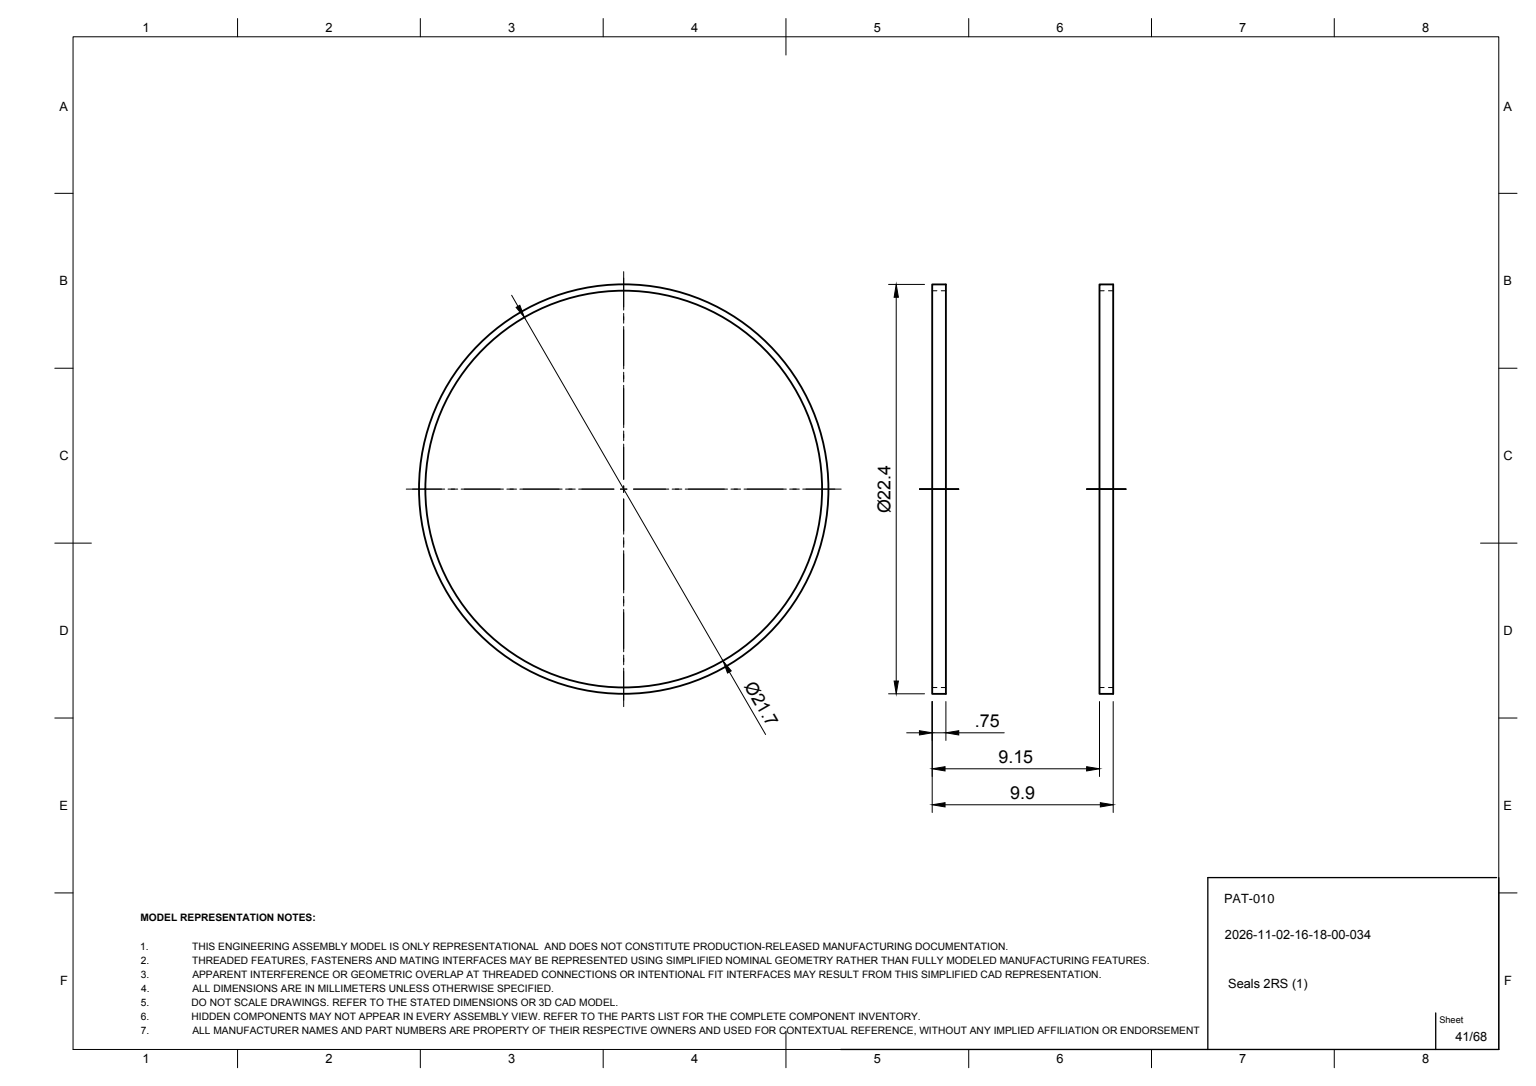
ISO-10303-21;
HEADER;
/* Generated by software containing ST-Developer
 * from STEP Tools, Inc. (www.steptools.com) 
 */

FILE_DESCRIPTION(
/* description */ ('Belt conveyor head drive unit'),
/* implementation_level */ '2;1');

FILE_NAME(
/* name */ 'Seals 2RS (1).step',
/* time_stamp */ '2026-10-28T03:26:19-07:00',
/* author */ (''),
/* organization */ (''),
/* preprocessor_version */ 'ST-DEVELOPER v20.2',
/* originating_system */ 'Autodesk Translation Framework v15.17.0.0',
/* authorisation */ '');

FILE_SCHEMA (('AUTOMOTIVE_DESIGN { 1 0 10303 214 3 1 1 }'));
ENDSEC;

DATA;
#10=MECHANICAL_DESIGN_GEOMETRIC_PRESENTATION_REPRESENTATION('',(#898,#899),#27069);
#746=SHAPE_REPRESENTATION_RELATIONSHIP('SRR','None',#27392,#815);
#815=ADVANCED_BREP_SHAPE_REPRESENTATION('',(#982,#983),#27034);
#898=STYLED_ITEM('',(#27797),#982);
#899=STYLED_ITEM('',(#27797),#983);
#982=MANIFOLD_SOLID_BREP('Body1',#13764);
#983=MANIFOLD_SOLID_BREP('Body2',#13765);
#1167=FACE_BOUND('',#3001,.T.);
#1168=FACE_BOUND('',#3004,.T.);
#1169=FACE_BOUND('',#3007,.T.);
#1170=FACE_BOUND('',#3010,.T.);
#1478=PLANE('',#15460);
#1479=PLANE('',#15465);
#1480=PLANE('',#15468);
#1481=PLANE('',#15473);
#2045=FACE_OUTER_BOUND('',#3000,.T.);
#2046=FACE_OUTER_BOUND('',#3002,.T.);
#2047=FACE_OUTER_BOUND('',#3003,.T.);
#2048=FACE_OUTER_BOUND('',#3005,.T.);
#2049=FACE_OUTER_BOUND('',#3006,.T.);
#2050=FACE_OUTER_BOUND('',#3008,.T.);
#2051=FACE_OUTER_BOUND('',#3009,.T.);
#2052=FACE_OUTER_BOUND('',#3011,.T.);
#3000=EDGE_LOOP('',(#10728));
#3001=EDGE_LOOP('',(#10729));
#3002=EDGE_LOOP('',(#10730,#10731,#10732,#10733));
#3003=EDGE_LOOP('',(#10734));
#3004=EDGE_LOOP('',(#10735));
#3005=EDGE_LOOP('',(#10736,#10737,#10738,#10739));
#3006=EDGE_LOOP('',(#10740));
#3007=EDGE_LOOP('',(#10741));
#3008=EDGE_LOOP('',(#10742,#10743,#10744,#10745));
#3009=EDGE_LOOP('',(#10746));
#3010=EDGE_LOOP('',(#10747));
#3011=EDGE_LOOP('',(#10748,#10749,#10750,#10751));
#3912=LINE('',#23560,#4704);
#3913=LINE('',#23565,#4705);
#3914=LINE('',#23574,#4706);
#3915=LINE('',#23579,#4707);
#4704=VECTOR('',#18654,1.119765);
#4705=VECTOR('',#18661,1.085235);
#4706=VECTOR('',#18672,1.119765);
#4707=VECTOR('',#18679,1.085235);
#5521=CIRCLE('',#15461,1.119765);
#5522=CIRCLE('',#15462,1.085235);
#5523=CIRCLE('',#15464,1.119765);
#5524=CIRCLE('',#15466,1.085235);
#5525=CIRCLE('',#15469,1.119765);
#5526=CIRCLE('',#15470,1.085235);
#5527=CIRCLE('',#15472,1.119765);
#5528=CIRCLE('',#15474,1.085235);
#6559=VERTEX_POINT('',#23553);
#6560=VERTEX_POINT('',#23555);
#6561=VERTEX_POINT('',#23558);
#6562=VERTEX_POINT('',#23562);
#6563=VERTEX_POINT('',#23567);
#6564=VERTEX_POINT('',#23569);
#6565=VERTEX_POINT('',#23572);
#6566=VERTEX_POINT('',#23576);
#8056=EDGE_CURVE('',#6559,#6559,#5521,.T.);
#8057=EDGE_CURVE('',#6560,#6560,#5522,.T.);
#8058=EDGE_CURVE('',#6561,#6561,#5523,.T.);
#8059=EDGE_CURVE('',#6561,#6559,#3912,.T.);
#8060=EDGE_CURVE('',#6562,#6562,#5524,.T.);
#8061=EDGE_CURVE('',#6562,#6560,#3913,.T.);
#8062=EDGE_CURVE('',#6563,#6563,#5525,.T.);
#8063=EDGE_CURVE('',#6564,#6564,#5526,.T.);
#8064=EDGE_CURVE('',#6565,#6565,#5527,.T.);
#8065=EDGE_CURVE('',#6565,#6563,#3914,.T.);
#8066=EDGE_CURVE('',#6566,#6566,#5528,.T.);
#8067=EDGE_CURVE('',#6566,#6564,#3915,.T.);
#10728=ORIENTED_EDGE('',*,*,#8056,.F.);
#10729=ORIENTED_EDGE('',*,*,#8057,.T.);
#10730=ORIENTED_EDGE('',*,*,#8058,.F.);
#10731=ORIENTED_EDGE('',*,*,#8059,.T.);
#10732=ORIENTED_EDGE('',*,*,#8056,.T.);
#10733=ORIENTED_EDGE('',*,*,#8059,.F.);
#10734=ORIENTED_EDGE('',*,*,#8058,.T.);
#10735=ORIENTED_EDGE('',*,*,#8060,.F.);
#10736=ORIENTED_EDGE('',*,*,#8060,.T.);
#10737=ORIENTED_EDGE('',*,*,#8061,.T.);
#10738=ORIENTED_EDGE('',*,*,#8057,.F.);
#10739=ORIENTED_EDGE('',*,*,#8061,.F.);
#10740=ORIENTED_EDGE('',*,*,#8062,.F.);
#10741=ORIENTED_EDGE('',*,*,#8063,.T.);
#10742=ORIENTED_EDGE('',*,*,#8064,.F.);
#10743=ORIENTED_EDGE('',*,*,#8065,.T.);
#10744=ORIENTED_EDGE('',*,*,#8062,.T.);
#10745=ORIENTED_EDGE('',*,*,#8065,.F.);
#10746=ORIENTED_EDGE('',*,*,#8064,.T.);
#10747=ORIENTED_EDGE('',*,*,#8066,.F.);
#10748=ORIENTED_EDGE('',*,*,#8066,.T.);
#10749=ORIENTED_EDGE('',*,*,#8067,.T.);
#10750=ORIENTED_EDGE('',*,*,#8063,.F.);
#10751=ORIENTED_EDGE('',*,*,#8067,.F.);
#12697=CYLINDRICAL_SURFACE('',#15463,1.119765);
#12698=CYLINDRICAL_SURFACE('',#15467,1.085235);
#12699=CYLINDRICAL_SURFACE('',#15471,1.119765);
#12700=CYLINDRICAL_SURFACE('',#15475,1.085235);
#13324=ADVANCED_FACE('',(#2045,#1167),#1478,.T.);
#13325=ADVANCED_FACE('',(#2046),#12697,.T.);
#13326=ADVANCED_FACE('',(#2047,#1168),#1479,.T.);
#13327=ADVANCED_FACE('',(#2048),#12698,.F.);
#13328=ADVANCED_FACE('',(#2049,#1169),#1480,.T.);
#13329=ADVANCED_FACE('',(#2050),#12699,.T.);
#13330=ADVANCED_FACE('',(#2051,#1170),#1481,.T.);
#13331=ADVANCED_FACE('',(#2052),#12700,.F.);
#13764=CLOSED_SHELL('',(#13324,#13325,#13326,#13327));
#13765=CLOSED_SHELL('',(#13328,#13329,#13330,#13331));
#15459=AXIS2_PLACEMENT_3D('',#23551,#18642,#18643);
#15460=AXIS2_PLACEMENT_3D('',#23552,#18644,#18645);
#15461=AXIS2_PLACEMENT_3D('',#23554,#18646,#18647);
#15462=AXIS2_PLACEMENT_3D('',#23556,#18648,#18649);
#15463=AXIS2_PLACEMENT_3D('',#23557,#18650,#18651);
#15464=AXIS2_PLACEMENT_3D('',#23559,#18652,#18653);
#15465=AXIS2_PLACEMENT_3D('',#23561,#18655,#18656);
#15466=AXIS2_PLACEMENT_3D('',#23563,#18657,#18658);
#15467=AXIS2_PLACEMENT_3D('',#23564,#18659,#18660);
#15468=AXIS2_PLACEMENT_3D('',#23566,#18662,#18663);
#15469=AXIS2_PLACEMENT_3D('',#23568,#18664,#18665);
#15470=AXIS2_PLACEMENT_3D('',#23570,#18666,#18667);
#15471=AXIS2_PLACEMENT_3D('',#23571,#18668,#18669);
#15472=AXIS2_PLACEMENT_3D('',#23573,#18670,#18671);
#15473=AXIS2_PLACEMENT_3D('',#23575,#18673,#18674);
#15474=AXIS2_PLACEMENT_3D('',#23577,#18675,#18676);
#15475=AXIS2_PLACEMENT_3D('',#23578,#18677,#18678);
#18642=DIRECTION('axis',(0.,0.,1.));
#18643=DIRECTION('refdir',(1.,0.,0.));
#18644=DIRECTION('center_axis',(0.,1.,0.));
#18645=DIRECTION('ref_axis',(0.,0.,1.));
#18646=DIRECTION('center_axis',(0.,-1.,0.));
#18647=DIRECTION('ref_axis',(1.,0.,0.));
#18648=DIRECTION('center_axis',(0.,-1.,0.));
#18649=DIRECTION('ref_axis',(1.,0.,0.));
#18650=DIRECTION('center_axis',(0.,-1.,0.));
#18651=DIRECTION('ref_axis',(1.,0.,0.));
#18652=DIRECTION('center_axis',(0.,-1.,0.));
#18653=DIRECTION('ref_axis',(1.,0.,0.));
#18654=DIRECTION('',(0.,1.,0.));
#18655=DIRECTION('center_axis',(0.,-1.,0.));
#18656=DIRECTION('ref_axis',(0.,0.,-1.));
#18657=DIRECTION('center_axis',(0.,-1.,0.));
#18658=DIRECTION('ref_axis',(1.,0.,0.));
#18659=DIRECTION('center_axis',(0.,-1.,0.));
#18660=DIRECTION('ref_axis',(1.,0.,0.));
#18661=DIRECTION('',(0.,1.,0.));
#18662=DIRECTION('center_axis',(0.,1.,0.));
#18663=DIRECTION('ref_axis',(0.,0.,1.));
#18664=DIRECTION('center_axis',(0.,-1.,0.));
#18665=DIRECTION('ref_axis',(1.,0.,0.));
#18666=DIRECTION('center_axis',(0.,-1.,0.));
#18667=DIRECTION('ref_axis',(1.,0.,0.));
#18668=DIRECTION('center_axis',(0.,-1.,0.));
#18669=DIRECTION('ref_axis',(1.,0.,0.));
#18670=DIRECTION('center_axis',(0.,-1.,0.));
#18671=DIRECTION('ref_axis',(1.,0.,0.));
#18672=DIRECTION('',(0.,1.,0.));
#18673=DIRECTION('center_axis',(0.,-1.,0.));
#18674=DIRECTION('ref_axis',(0.,0.,-1.));
#18675=DIRECTION('center_axis',(0.,-1.,0.));
#18676=DIRECTION('ref_axis',(1.,0.,0.));
#18677=DIRECTION('center_axis',(0.,-1.,0.));
#18678=DIRECTION('ref_axis',(1.,0.,0.));
#18679=DIRECTION('',(0.,1.,0.));
#23551=CARTESIAN_POINT('',(0.,0.,0.));
#23552=CARTESIAN_POINT('Origin',(1.119765,0.495,0.));
#23553=CARTESIAN_POINT('',(-1.119765,0.495,-1.37131662304724E-16));
#23554=CARTESIAN_POINT('Origin',(0.,0.495,0.));
#23555=CARTESIAN_POINT('',(-1.085235,0.495,-1.32902956907268E-16));
#23556=CARTESIAN_POINT('Origin',(0.,0.495,0.));
#23557=CARTESIAN_POINT('Origin',(0.,0.4575,0.));
#23558=CARTESIAN_POINT('',(-1.119765,0.42,-1.37131662304724E-16));
#23559=CARTESIAN_POINT('Origin',(0.,0.42,0.));
#23560=CARTESIAN_POINT('',(-1.119765,0.4575,-1.37131662304724E-16));
#23561=CARTESIAN_POINT('Origin',(1.085235,0.42,0.));
#23562=CARTESIAN_POINT('',(-1.085235,0.42,-1.32902956907268E-16));
#23563=CARTESIAN_POINT('Origin',(0.,0.42,0.));
#23564=CARTESIAN_POINT('Origin',(0.,0.4575,0.));
#23565=CARTESIAN_POINT('',(-1.085235,0.4575,-1.32902956907268E-16));
#23566=CARTESIAN_POINT('Origin',(1.119765,-0.42,0.));
#23567=CARTESIAN_POINT('',(-1.119765,-0.42,-1.37131662304724E-16));
#23568=CARTESIAN_POINT('Origin',(0.,-0.42,0.));
#23569=CARTESIAN_POINT('',(-1.085235,-0.42,-1.32902956907268E-16));
#23570=CARTESIAN_POINT('Origin',(0.,-0.42,0.));
#23571=CARTESIAN_POINT('Origin',(0.,-0.4575,0.));
#23572=CARTESIAN_POINT('',(-1.119765,-0.495,-1.37131662304724E-16));
#23573=CARTESIAN_POINT('Origin',(0.,-0.495,0.));
#23574=CARTESIAN_POINT('',(-1.119765,-0.4575,-1.37131662304724E-16));
#23575=CARTESIAN_POINT('Origin',(1.085235,-0.495,0.));
#23576=CARTESIAN_POINT('',(-1.085235,-0.495,-1.32902956907268E-16));
#23577=CARTESIAN_POINT('Origin',(0.,-0.495,0.));
#23578=CARTESIAN_POINT('Origin',(0.,-0.4575,0.));
#23579=CARTESIAN_POINT('',(-1.085235,-0.4575,-1.32902956907268E-16));
#26957=UNCERTAINTY_MEASURE_WITH_UNIT(LENGTH_MEASURE(0.001),#27070,
'DISTANCE_ACCURACY_VALUE',
'Maximum model space distance between geometric entities at asserted c
onnectivities');
#26992=UNCERTAINTY_MEASURE_WITH_UNIT(LENGTH_MEASURE(0.001),#27070,
'DISTANCE_ACCURACY_VALUE',
'Maximum model space distance between geometric entities at asserted c
onnectivities');
#27034=(
GEOMETRIC_REPRESENTATION_CONTEXT(3)
GLOBAL_UNCERTAINTY_ASSIGNED_CONTEXT((#26957))
GLOBAL_UNIT_ASSIGNED_CONTEXT((#27070,#27072,#27073))
REPRESENTATION_CONTEXT('','3D')
);
#27069=(
GEOMETRIC_REPRESENTATION_CONTEXT(3)
GLOBAL_UNCERTAINTY_ASSIGNED_CONTEXT((#26992))
GLOBAL_UNIT_ASSIGNED_CONTEXT((#27070,#27072,#27073))
REPRESENTATION_CONTEXT('','3D')
);
#27070=(
LENGTH_UNIT()
NAMED_UNIT(*)
SI_UNIT(.CENTI.,.METRE.)
);
#27072=(
NAMED_UNIT(*)
PLANE_ANGLE_UNIT()
SI_UNIT($,.RADIAN.)
);
#27073=(
NAMED_UNIT(*)
SI_UNIT($,.STERADIAN.)
SOLID_ANGLE_UNIT()
);
#27115=SHAPE_DEFINITION_REPRESENTATION(#27196,#27392);
#27196=PRODUCT_DEFINITION_SHAPE('',$,#27469);
#27392=SHAPE_REPRESENTATION('',(#15459),#27034);
#27427=PRODUCT_DEFINITION_CONTEXT('part definition',#27657,'design');
#27469=PRODUCT_DEFINITION('Seals 2RS (1)','Seals 2RS (1)',#27545,#27427);
#27545=PRODUCT_DEFINITION_FORMATION('',$,#27700);
#27657=APPLICATION_CONTEXT(
'Core Data for Automotive Mechanical Design Process');
#27658=PRODUCT_CONTEXT('part definition',#27657,'mechanical');
#27700=PRODUCT('Seals 2RS (1)','Seals 2RS (1)','Seals 2RS (1)',(#27658));
#27791=COLOUR_RGB('Grey',0.48,0.52,0.57);
#27792=FILL_AREA_STYLE_COLOUR('',#27791);
#27793=FILL_AREA_STYLE('',(#27792));
#27794=SURFACE_STYLE_FILL_AREA(#27793);
#27795=SURFACE_SIDE_STYLE('',(#27794));
#27796=SURFACE_STYLE_USAGE(.BOTH.,#27795);
#27797=PRESENTATION_STYLE_ASSIGNMENT((#27796));
ENDSEC;
END-ISO-10303-21;
